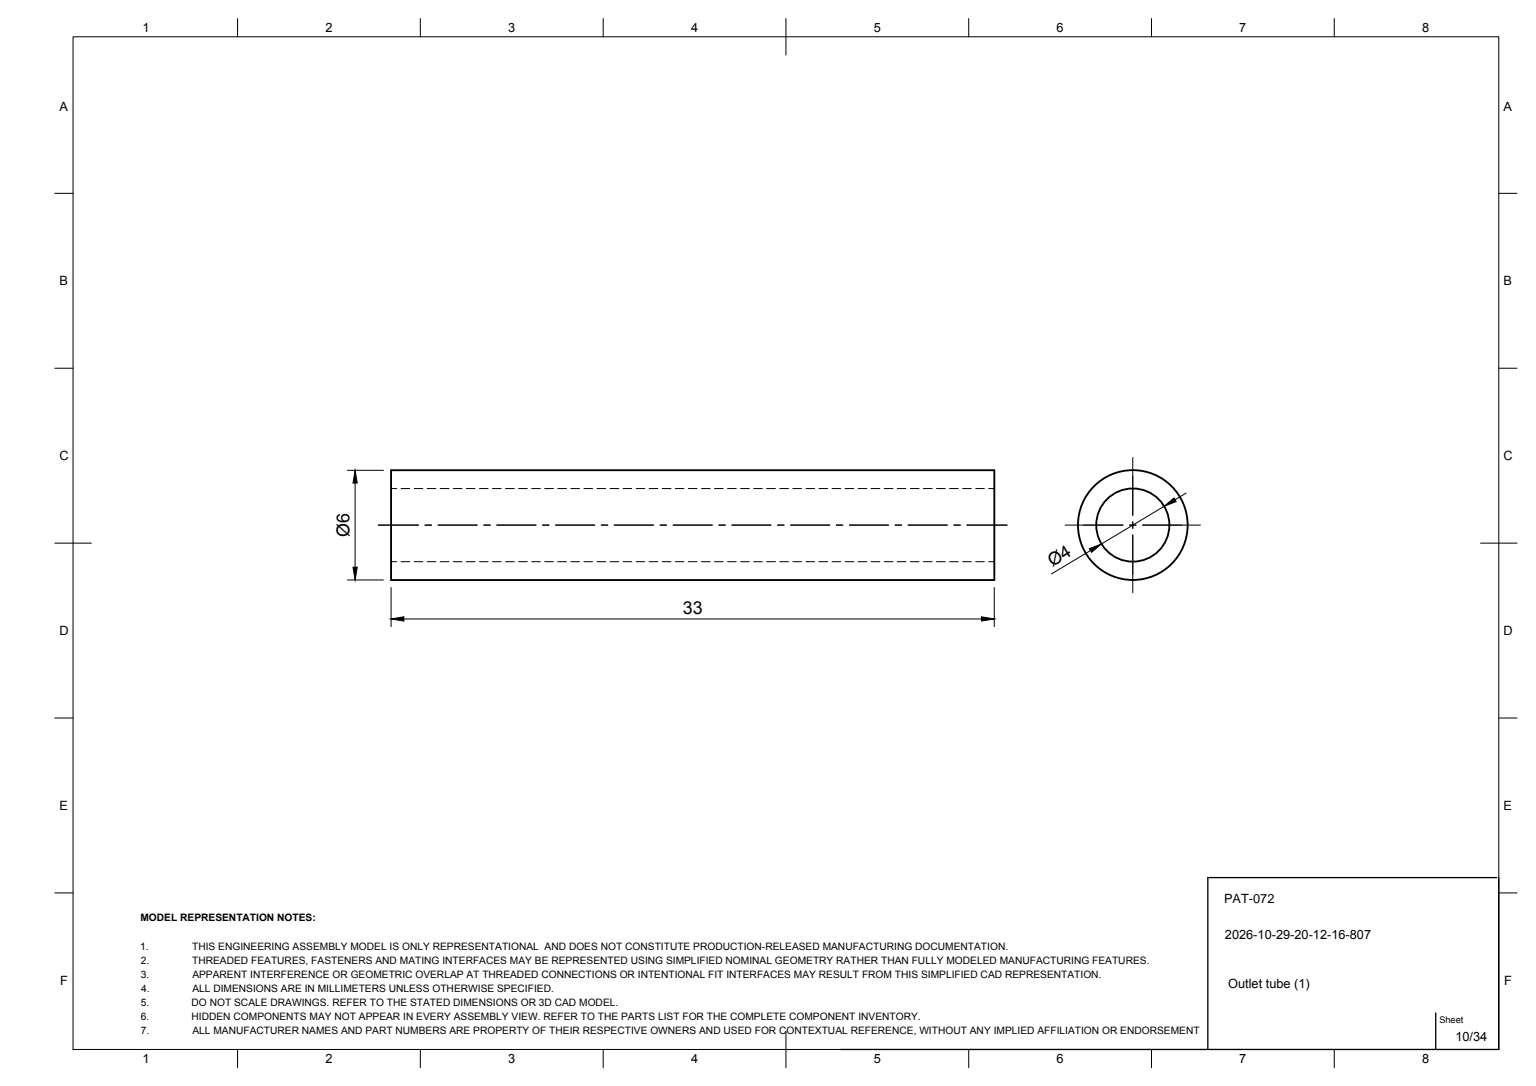
ISO-10303-21;
HEADER;
/* Generated by software containing ST-Developer
 * from STEP Tools, Inc. (www.steptools.com) 
 */

FILE_DESCRIPTION(
/* description */ ('PAT-072'),
/* implementation_level */ '2;1');

FILE_NAME(
/* name */ 'Outlet tube (1).step',
/* time_stamp */ '2026-10-29T20:11:56-07:00',
/* author */ (''),
/* organization */ (''),
/* preprocessor_version */ 'ST-DEVELOPER v20.2',
/* originating_system */ 'Autodesk Translation Framework v15.17.0.0',
/* authorisation */ '');

FILE_SCHEMA (('AUTOMOTIVE_DESIGN { 1 0 10303 214 3 1 1 }'));
ENDSEC;

DATA;
#10=MECHANICAL_DESIGN_GEOMETRIC_PRESENTATION_REPRESENTATION('',(#339),#11432);
#267=SHAPE_REPRESENTATION_RELATIONSHIP('SRR','None',#11571,#303);
#303=ADVANCED_BREP_SHAPE_REPRESENTATION('',(#375),#11402);
#339=STYLED_ITEM('',(#11812),#375);
#375=MANIFOLD_SOLID_BREP('Body1',#6074);
#466=FACE_BOUND('',#1347,.T.);
#467=FACE_BOUND('',#1349,.T.);
#629=PLANE('',#6731);
#630=PLANE('',#6732);
#908=FACE_OUTER_BOUND('',#1344,.T.);
#909=FACE_OUTER_BOUND('',#1345,.T.);
#910=FACE_OUTER_BOUND('',#1346,.T.);
#911=FACE_OUTER_BOUND('',#1348,.T.);
#1344=EDGE_LOOP('',(#4540,#4541,#4542,#4543));
#1345=EDGE_LOOP('',(#4544,#4545,#4546,#4547));
#1346=EDGE_LOOP('',(#4548));
#1347=EDGE_LOOP('',(#4549));
#1348=EDGE_LOOP('',(#4550));
#1349=EDGE_LOOP('',(#4551));
#1817=LINE('',#10046,#2236);
#1818=LINE('',#10052,#2237);
#2236=VECTOR('',#7818,0.2);
#2237=VECTOR('',#7825,0.3);
#2641=CIRCLE('',#6726,0.2);
#2642=CIRCLE('',#6727,0.2);
#2643=CIRCLE('',#6729,0.3);
#2644=CIRCLE('',#6730,0.3);
#2990=VERTEX_POINT('',#10043);
#2991=VERTEX_POINT('',#10045);
#2992=VERTEX_POINT('',#10049);
#2993=VERTEX_POINT('',#10051);
#3559=EDGE_CURVE('',#2990,#2990,#2641,.T.);
#3560=EDGE_CURVE('',#2990,#2991,#1817,.T.);
#3561=EDGE_CURVE('',#2991,#2991,#2642,.T.);
#3562=EDGE_CURVE('',#2992,#2992,#2643,.T.);
#3563=EDGE_CURVE('',#2992,#2993,#1818,.T.);
#3564=EDGE_CURVE('',#2993,#2993,#2644,.T.);
#4540=ORIENTED_EDGE('',*,*,#3559,.F.);
#4541=ORIENTED_EDGE('',*,*,#3560,.T.);
#4542=ORIENTED_EDGE('',*,*,#3561,.T.);
#4543=ORIENTED_EDGE('',*,*,#3560,.F.);
#4544=ORIENTED_EDGE('',*,*,#3562,.F.);
#4545=ORIENTED_EDGE('',*,*,#3563,.T.);
#4546=ORIENTED_EDGE('',*,*,#3564,.T.);
#4547=ORIENTED_EDGE('',*,*,#3563,.F.);
#4548=ORIENTED_EDGE('',*,*,#3562,.T.);
#4549=ORIENTED_EDGE('',*,*,#3559,.T.);
#4550=ORIENTED_EDGE('',*,*,#3564,.F.);
#4551=ORIENTED_EDGE('',*,*,#3561,.F.);
#5611=CYLINDRICAL_SURFACE('',#6725,0.2);
#5612=CYLINDRICAL_SURFACE('',#6728,0.3);
#5807=ADVANCED_FACE('',(#908),#5611,.F.);
#5808=ADVANCED_FACE('',(#909),#5612,.T.);
#5809=ADVANCED_FACE('',(#910,#466),#629,.T.);
#5810=ADVANCED_FACE('',(#911,#467),#630,.F.);
#6074=CLOSED_SHELL('',(#5807,#5808,#5809,#5810));
#6724=AXIS2_PLACEMENT_3D('',#10041,#7812,#7813);
#6725=AXIS2_PLACEMENT_3D('',#10042,#7814,#7815);
#6726=AXIS2_PLACEMENT_3D('',#10044,#7816,#7817);
#6727=AXIS2_PLACEMENT_3D('',#10047,#7819,#7820);
#6728=AXIS2_PLACEMENT_3D('',#10048,#7821,#7822);
#6729=AXIS2_PLACEMENT_3D('',#10050,#7823,#7824);
#6730=AXIS2_PLACEMENT_3D('',#10053,#7826,#7827);
#6731=AXIS2_PLACEMENT_3D('',#10054,#7828,#7829);
#6732=AXIS2_PLACEMENT_3D('',#10055,#7830,#7831);
#7812=DIRECTION('axis',(0.,0.,1.));
#7813=DIRECTION('refdir',(1.,0.,0.));
#7814=DIRECTION('center_axis',(0.,1.,0.));
#7815=DIRECTION('ref_axis',(1.,0.,0.));
#7816=DIRECTION('center_axis',(0.,-1.,0.));
#7817=DIRECTION('ref_axis',(1.,0.,0.));
#7818=DIRECTION('',(0.,-1.,0.));
#7819=DIRECTION('center_axis',(0.,-1.,0.));
#7820=DIRECTION('ref_axis',(1.,0.,0.));
#7821=DIRECTION('center_axis',(0.,1.,0.));
#7822=DIRECTION('ref_axis',(1.,0.,0.));
#7823=DIRECTION('center_axis',(0.,1.,0.));
#7824=DIRECTION('ref_axis',(1.,0.,0.));
#7825=DIRECTION('',(0.,-1.,0.));
#7826=DIRECTION('center_axis',(0.,1.,0.));
#7827=DIRECTION('ref_axis',(1.,0.,0.));
#7828=DIRECTION('center_axis',(0.,1.,0.));
#7829=DIRECTION('ref_axis',(1.,0.,0.));
#7830=DIRECTION('center_axis',(0.,1.,0.));
#7831=DIRECTION('ref_axis',(1.,0.,0.));
#10041=CARTESIAN_POINT('',(0.,0.,0.));
#10042=CARTESIAN_POINT('Origin',(-1.25,-6.5,4.));
#10043=CARTESIAN_POINT('',(-1.45,-3.2,4.));
#10044=CARTESIAN_POINT('Origin',(-1.25,-3.2,4.));
#10045=CARTESIAN_POINT('',(-1.45,-6.5,4.));
#10046=CARTESIAN_POINT('',(-1.45,-6.5,4.));
#10047=CARTESIAN_POINT('Origin',(-1.25,-6.5,4.));
#10048=CARTESIAN_POINT('Origin',(-1.25,-6.5,4.));
#10049=CARTESIAN_POINT('',(-1.55,-3.2,4.));
#10050=CARTESIAN_POINT('Origin',(-1.25,-3.2,4.));
#10051=CARTESIAN_POINT('',(-1.55,-6.5,4.));
#10052=CARTESIAN_POINT('',(-1.55,-6.5,4.));
#10053=CARTESIAN_POINT('Origin',(-1.25,-6.5,4.));
#10054=CARTESIAN_POINT('Origin',(-1.25,-3.2,4.));
#10055=CARTESIAN_POINT('Origin',(-1.25,-6.5,4.));
#11363=UNCERTAINTY_MEASURE_WITH_UNIT(LENGTH_MEASURE(0.001),#11433,
'DISTANCE_ACCURACY_VALUE',
'Maximum model space distance between geometric entities at asserted c
onnectivities');
#11393=UNCERTAINTY_MEASURE_WITH_UNIT(LENGTH_MEASURE(0.001),#11433,
'DISTANCE_ACCURACY_VALUE',
'Maximum model space distance between geometric entities at asserted c
onnectivities');
#11402=(
GEOMETRIC_REPRESENTATION_CONTEXT(3)
GLOBAL_UNCERTAINTY_ASSIGNED_CONTEXT((#11363))
GLOBAL_UNIT_ASSIGNED_CONTEXT((#11433,#11435,#11436))
REPRESENTATION_CONTEXT('','3D')
);
#11432=(
GEOMETRIC_REPRESENTATION_CONTEXT(3)
GLOBAL_UNCERTAINTY_ASSIGNED_CONTEXT((#11393))
GLOBAL_UNIT_ASSIGNED_CONTEXT((#11433,#11435,#11436))
REPRESENTATION_CONTEXT('','3D')
);
#11433=(
LENGTH_UNIT()
NAMED_UNIT(*)
SI_UNIT(.CENTI.,.METRE.)
);
#11435=(
NAMED_UNIT(*)
PLANE_ANGLE_UNIT()
SI_UNIT($,.RADIAN.)
);
#11436=(
NAMED_UNIT(*)
SI_UNIT($,.STERADIAN.)
SOLID_ANGLE_UNIT()
);
#11445=SHAPE_DEFINITION_REPRESENTATION(#11483,#11571);
#11483=PRODUCT_DEFINITION_SHAPE('',$,#11610);
#11571=SHAPE_REPRESENTATION('',(#6724),#11402);
#11601=PRODUCT_DEFINITION_CONTEXT('part definition',#11717,'design');
#11610=PRODUCT_DEFINITION('Outlet tube (1)','Outlet tube (1)',
#11648,#11601);
#11648=PRODUCT_DEFINITION_FORMATION('',$,#11727);
#11717=APPLICATION_CONTEXT(
'Core Data for Automotive Mechanical Design Process');
#11718=PRODUCT_CONTEXT('part definition',#11717,'mechanical');
#11727=PRODUCT('Outlet tube (1)','Outlet tube (1)',
'Outlet tube (1)',(#11718));
#11806=COLOUR_RGB('Sky Blue',0.24,0.69,0.87);
#11807=FILL_AREA_STYLE_COLOUR('',#11806);
#11808=FILL_AREA_STYLE('',(#11807));
#11809=SURFACE_STYLE_FILL_AREA(#11808);
#11810=SURFACE_SIDE_STYLE('',(#11809));
#11811=SURFACE_STYLE_USAGE(.BOTH.,#11810);
#11812=PRESENTATION_STYLE_ASSIGNMENT((#11811));
ENDSEC;
END-ISO-10303-21;
